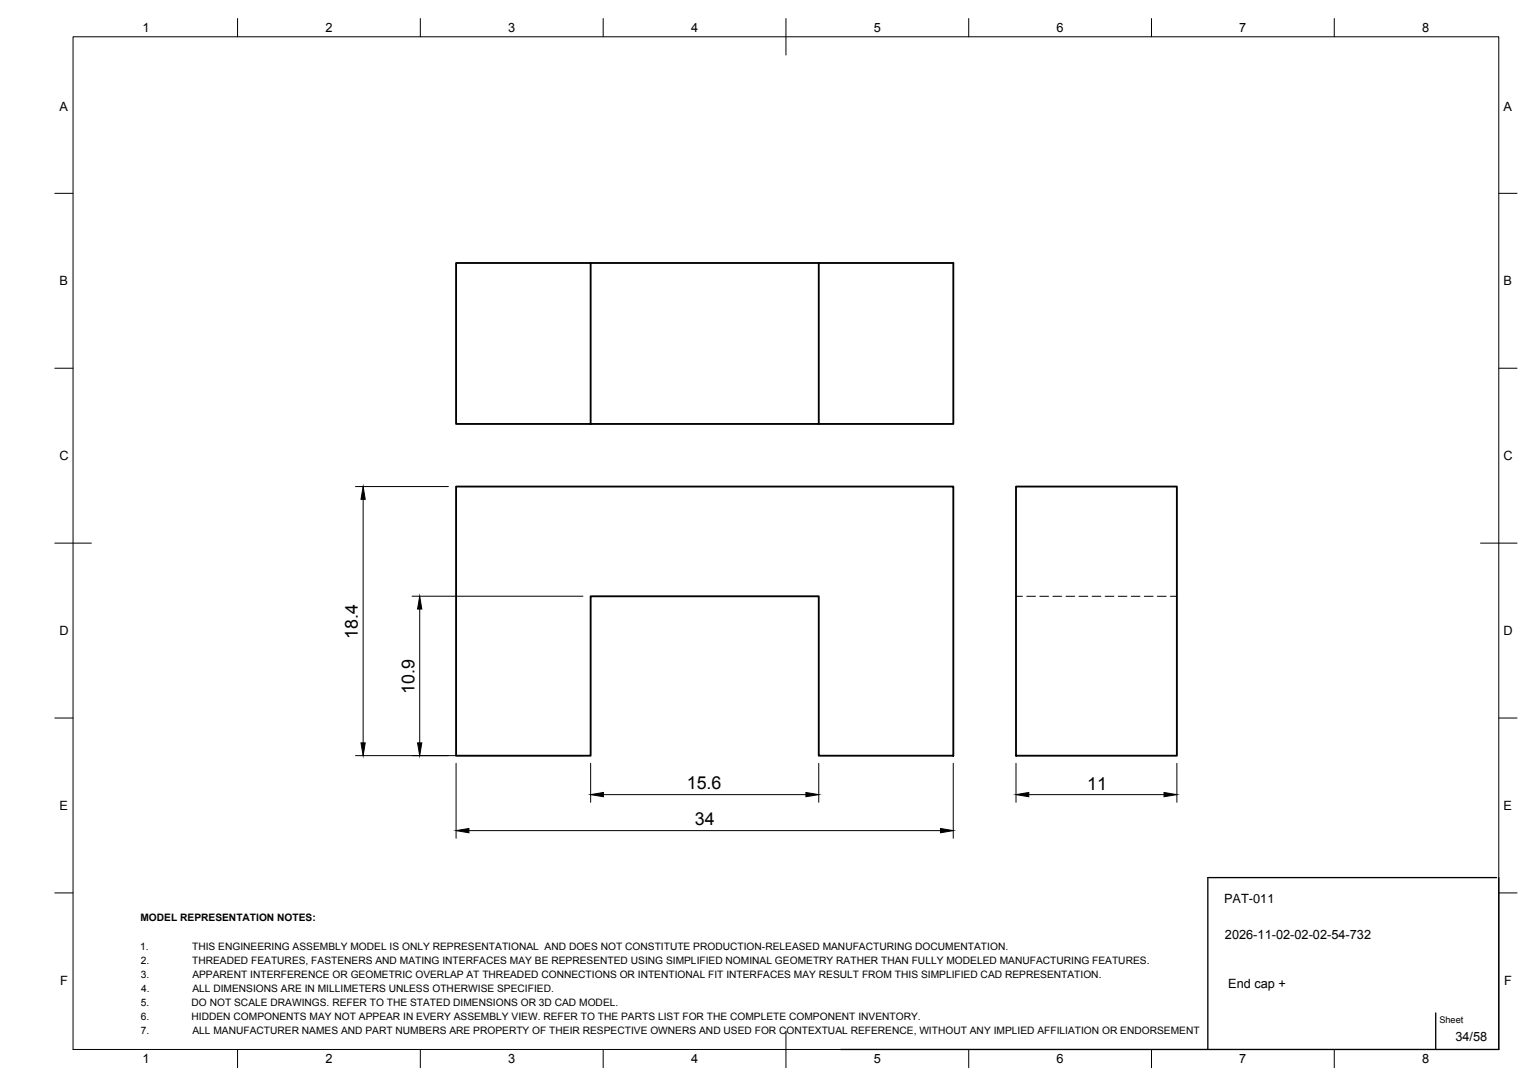
ISO-10303-21;
HEADER;
/* Generated by software containing ST-Developer
 * from STEP Tools, Inc. (www.steptools.com) 
 */

FILE_DESCRIPTION(
/* description */ ('Belt tension measurement rig'),
/* implementation_level */ '2;1');

FILE_NAME(
/* name */ 'End cap +.step',
/* time_stamp */ '2026-10-28T03:24:44-07:00',
/* author */ (''),
/* organization */ (''),
/* preprocessor_version */ 'ST-DEVELOPER v20.2',
/* originating_system */ 'Autodesk Translation Framework v15.17.0.0',
/* authorisation */ '');

FILE_SCHEMA (('AUTOMOTIVE_DESIGN { 1 0 10303 214 3 1 1 }'));
ENDSEC;

DATA;
#10=MECHANICAL_DESIGN_GEOMETRIC_PRESENTATION_REPRESENTATION('',(#728),#23587);
#610=SHAPE_REPRESENTATION_RELATIONSHIP('SRR','None',#23858,#665);
#665=ADVANCED_BREP_SHAPE_REPRESENTATION('',(#798),#23556);
#728=STYLED_ITEM('',(#24204),#798);
#798=MANIFOLD_SOLID_BREP('Body1',#12233);
#1219=PLANE('',#13605);
#1220=PLANE('',#13606);
#1221=PLANE('',#13607);
#1222=PLANE('',#13608);
#1223=PLANE('',#13609);
#1224=PLANE('',#13610);
#1225=PLANE('',#13611);
#1226=PLANE('',#13612);
#1227=PLANE('',#13613);
#1228=PLANE('',#13614);
#1699=FACE_OUTER_BOUND('',#2547,.T.);
#1700=FACE_OUTER_BOUND('',#2548,.T.);
#1701=FACE_OUTER_BOUND('',#2549,.T.);
#1702=FACE_OUTER_BOUND('',#2550,.T.);
#1703=FACE_OUTER_BOUND('',#2551,.T.);
#1704=FACE_OUTER_BOUND('',#2552,.T.);
#1705=FACE_OUTER_BOUND('',#2553,.T.);
#1706=FACE_OUTER_BOUND('',#2554,.T.);
#1707=FACE_OUTER_BOUND('',#2555,.T.);
#1708=FACE_OUTER_BOUND('',#2556,.T.);
#2547=EDGE_LOOP('',(#9506,#9507,#9508,#9509));
#2548=EDGE_LOOP('',(#9510,#9511,#9512,#9513));
#2549=EDGE_LOOP('',(#9514,#9515,#9516,#9517));
#2550=EDGE_LOOP('',(#9518,#9519,#9520,#9521));
#2551=EDGE_LOOP('',(#9522,#9523,#9524,#9525));
#2552=EDGE_LOOP('',(#9526,#9527,#9528,#9529));
#2553=EDGE_LOOP('',(#9530,#9531,#9532,#9533));
#2554=EDGE_LOOP('',(#9534,#9535,#9536,#9537));
#2555=EDGE_LOOP('',(#9538,#9539,#9540,#9541,#9542,#9543,#9544,#9545));
#2556=EDGE_LOOP('',(#9546,#9547,#9548,#9549,#9550,#9551,#9552,#9553));
#3383=LINE('',#20682,#4134);
#3384=LINE('',#20684,#4135);
#3385=LINE('',#20686,#4136);
#3386=LINE('',#20687,#4137);
#3387=LINE('',#20690,#4138);
#3388=LINE('',#20692,#4139);
#3389=LINE('',#20693,#4140);
#3390=LINE('',#20696,#4141);
#3391=LINE('',#20698,#4142);
#3392=LINE('',#20699,#4143);
#3393=LINE('',#20702,#4144);
#3394=LINE('',#20704,#4145);
#3395=LINE('',#20705,#4146);
#3396=LINE('',#20708,#4147);
#3397=LINE('',#20710,#4148);
#3398=LINE('',#20711,#4149);
#3399=LINE('',#20714,#4150);
#3400=LINE('',#20716,#4151);
#3401=LINE('',#20717,#4152);
#3402=LINE('',#20720,#4153);
#3403=LINE('',#20722,#4154);
#3404=LINE('',#20723,#4155);
#3405=LINE('',#20725,#4156);
#3406=LINE('',#20726,#4157);
#4134=VECTOR('',#16392,1.);
#4135=VECTOR('',#16393,1.);
#4136=VECTOR('',#16394,1.);
#4137=VECTOR('',#16395,1.);
#4138=VECTOR('',#16398,1.);
#4139=VECTOR('',#16399,1.);
#4140=VECTOR('',#16400,1.);
#4141=VECTOR('',#16403,1.);
#4142=VECTOR('',#16404,1.);
#4143=VECTOR('',#16405,1.);
#4144=VECTOR('',#16408,1.);
#4145=VECTOR('',#16409,1.);
#4146=VECTOR('',#16410,1.);
#4147=VECTOR('',#16413,1.);
#4148=VECTOR('',#16414,1.);
#4149=VECTOR('',#16415,1.);
#4150=VECTOR('',#16418,1.);
#4151=VECTOR('',#16419,1.);
#4152=VECTOR('',#16420,1.);
#4153=VECTOR('',#16423,1.);
#4154=VECTOR('',#16424,1.);
#4155=VECTOR('',#16425,1.);
#4156=VECTOR('',#16428,1.);
#4157=VECTOR('',#16429,1.);
#5767=VERTEX_POINT('',#20680);
#5768=VERTEX_POINT('',#20681);
#5769=VERTEX_POINT('',#20683);
#5770=VERTEX_POINT('',#20685);
#5771=VERTEX_POINT('',#20689);
#5772=VERTEX_POINT('',#20691);
#5773=VERTEX_POINT('',#20695);
#5774=VERTEX_POINT('',#20697);
#5775=VERTEX_POINT('',#20701);
#5776=VERTEX_POINT('',#20703);
#5777=VERTEX_POINT('',#20707);
#5778=VERTEX_POINT('',#20709);
#5779=VERTEX_POINT('',#20713);
#5780=VERTEX_POINT('',#20715);
#5781=VERTEX_POINT('',#20719);
#5782=VERTEX_POINT('',#20721);
#7112=EDGE_CURVE('',#5767,#5768,#3383,.T.);
#7113=EDGE_CURVE('',#5768,#5769,#3384,.T.);
#7114=EDGE_CURVE('',#5770,#5769,#3385,.T.);
#7115=EDGE_CURVE('',#5767,#5770,#3386,.T.);
#7116=EDGE_CURVE('',#5771,#5767,#3387,.T.);
#7117=EDGE_CURVE('',#5772,#5770,#3388,.T.);
#7118=EDGE_CURVE('',#5771,#5772,#3389,.T.);
#7119=EDGE_CURVE('',#5773,#5771,#3390,.T.);
#7120=EDGE_CURVE('',#5774,#5772,#3391,.T.);
#7121=EDGE_CURVE('',#5773,#5774,#3392,.T.);
#7122=EDGE_CURVE('',#5775,#5773,#3393,.T.);
#7123=EDGE_CURVE('',#5776,#5774,#3394,.T.);
#7124=EDGE_CURVE('',#5775,#5776,#3395,.T.);
#7125=EDGE_CURVE('',#5777,#5775,#3396,.T.);
#7126=EDGE_CURVE('',#5778,#5776,#3397,.T.);
#7127=EDGE_CURVE('',#5777,#5778,#3398,.T.);
#7128=EDGE_CURVE('',#5779,#5777,#3399,.T.);
#7129=EDGE_CURVE('',#5780,#5778,#3400,.T.);
#7130=EDGE_CURVE('',#5779,#5780,#3401,.T.);
#7131=EDGE_CURVE('',#5781,#5779,#3402,.T.);
#7132=EDGE_CURVE('',#5782,#5780,#3403,.T.);
#7133=EDGE_CURVE('',#5781,#5782,#3404,.T.);
#7134=EDGE_CURVE('',#5768,#5781,#3405,.T.);
#7135=EDGE_CURVE('',#5769,#5782,#3406,.T.);
#9506=ORIENTED_EDGE('',*,*,#7112,.T.);
#9507=ORIENTED_EDGE('',*,*,#7113,.T.);
#9508=ORIENTED_EDGE('',*,*,#7114,.F.);
#9509=ORIENTED_EDGE('',*,*,#7115,.F.);
#9510=ORIENTED_EDGE('',*,*,#7116,.T.);
#9511=ORIENTED_EDGE('',*,*,#7115,.T.);
#9512=ORIENTED_EDGE('',*,*,#7117,.F.);
#9513=ORIENTED_EDGE('',*,*,#7118,.F.);
#9514=ORIENTED_EDGE('',*,*,#7119,.T.);
#9515=ORIENTED_EDGE('',*,*,#7118,.T.);
#9516=ORIENTED_EDGE('',*,*,#7120,.F.);
#9517=ORIENTED_EDGE('',*,*,#7121,.F.);
#9518=ORIENTED_EDGE('',*,*,#7122,.T.);
#9519=ORIENTED_EDGE('',*,*,#7121,.T.);
#9520=ORIENTED_EDGE('',*,*,#7123,.F.);
#9521=ORIENTED_EDGE('',*,*,#7124,.F.);
#9522=ORIENTED_EDGE('',*,*,#7125,.T.);
#9523=ORIENTED_EDGE('',*,*,#7124,.T.);
#9524=ORIENTED_EDGE('',*,*,#7126,.F.);
#9525=ORIENTED_EDGE('',*,*,#7127,.F.);
#9526=ORIENTED_EDGE('',*,*,#7128,.T.);
#9527=ORIENTED_EDGE('',*,*,#7127,.T.);
#9528=ORIENTED_EDGE('',*,*,#7129,.F.);
#9529=ORIENTED_EDGE('',*,*,#7130,.F.);
#9530=ORIENTED_EDGE('',*,*,#7131,.T.);
#9531=ORIENTED_EDGE('',*,*,#7130,.T.);
#9532=ORIENTED_EDGE('',*,*,#7132,.F.);
#9533=ORIENTED_EDGE('',*,*,#7133,.F.);
#9534=ORIENTED_EDGE('',*,*,#7134,.T.);
#9535=ORIENTED_EDGE('',*,*,#7133,.T.);
#9536=ORIENTED_EDGE('',*,*,#7135,.F.);
#9537=ORIENTED_EDGE('',*,*,#7113,.F.);
#9538=ORIENTED_EDGE('',*,*,#7135,.T.);
#9539=ORIENTED_EDGE('',*,*,#7132,.T.);
#9540=ORIENTED_EDGE('',*,*,#7129,.T.);
#9541=ORIENTED_EDGE('',*,*,#7126,.T.);
#9542=ORIENTED_EDGE('',*,*,#7123,.T.);
#9543=ORIENTED_EDGE('',*,*,#7120,.T.);
#9544=ORIENTED_EDGE('',*,*,#7117,.T.);
#9545=ORIENTED_EDGE('',*,*,#7114,.T.);
#9546=ORIENTED_EDGE('',*,*,#7134,.F.);
#9547=ORIENTED_EDGE('',*,*,#7112,.F.);
#9548=ORIENTED_EDGE('',*,*,#7116,.F.);
#9549=ORIENTED_EDGE('',*,*,#7119,.F.);
#9550=ORIENTED_EDGE('',*,*,#7122,.F.);
#9551=ORIENTED_EDGE('',*,*,#7125,.F.);
#9552=ORIENTED_EDGE('',*,*,#7128,.F.);
#9553=ORIENTED_EDGE('',*,*,#7131,.F.);
#11840=ADVANCED_FACE('',(#1699),#1219,.T.);
#11841=ADVANCED_FACE('',(#1700),#1220,.T.);
#11842=ADVANCED_FACE('',(#1701),#1221,.T.);
#11843=ADVANCED_FACE('',(#1702),#1222,.T.);
#11844=ADVANCED_FACE('',(#1703),#1223,.T.);
#11845=ADVANCED_FACE('',(#1704),#1224,.T.);
#11846=ADVANCED_FACE('',(#1705),#1225,.T.);
#11847=ADVANCED_FACE('',(#1706),#1226,.T.);
#11848=ADVANCED_FACE('',(#1707),#1227,.T.);
#11849=ADVANCED_FACE('',(#1708),#1228,.F.);
#12233=CLOSED_SHELL('',(#11840,#11841,#11842,#11843,#11844,#11845,#11846,
#11847,#11848,#11849));
#13604=AXIS2_PLACEMENT_3D('',#20678,#16388,#16389);
#13605=AXIS2_PLACEMENT_3D('',#20679,#16390,#16391);
#13606=AXIS2_PLACEMENT_3D('',#20688,#16396,#16397);
#13607=AXIS2_PLACEMENT_3D('',#20694,#16401,#16402);
#13608=AXIS2_PLACEMENT_3D('',#20700,#16406,#16407);
#13609=AXIS2_PLACEMENT_3D('',#20706,#16411,#16412);
#13610=AXIS2_PLACEMENT_3D('',#20712,#16416,#16417);
#13611=AXIS2_PLACEMENT_3D('',#20718,#16421,#16422);
#13612=AXIS2_PLACEMENT_3D('',#20724,#16426,#16427);
#13613=AXIS2_PLACEMENT_3D('',#20727,#16430,#16431);
#13614=AXIS2_PLACEMENT_3D('',#20728,#16432,#16433);
#16388=DIRECTION('axis',(0.,0.,1.));
#16389=DIRECTION('refdir',(1.,0.,0.));
#16390=DIRECTION('center_axis',(0.,0.,1.));
#16391=DIRECTION('ref_axis',(0.,-1.,0.));
#16392=DIRECTION('',(0.,-1.,0.));
#16393=DIRECTION('',(1.,0.,0.));
#16394=DIRECTION('',(0.,-1.,0.));
#16395=DIRECTION('',(1.,0.,0.));
#16396=DIRECTION('center_axis',(0.,1.,0.));
#16397=DIRECTION('ref_axis',(0.,0.,1.));
#16398=DIRECTION('',(0.,0.,1.));
#16399=DIRECTION('',(0.,0.,1.));
#16400=DIRECTION('',(1.,0.,0.));
#16401=DIRECTION('center_axis',(0.,0.,-1.));
#16402=DIRECTION('ref_axis',(0.,1.,0.));
#16403=DIRECTION('',(0.,1.,0.));
#16404=DIRECTION('',(0.,1.,0.));
#16405=DIRECTION('',(1.,0.,0.));
#16406=DIRECTION('center_axis',(0.,-1.,0.));
#16407=DIRECTION('ref_axis',(0.,0.,-1.));
#16408=DIRECTION('',(0.,0.,-1.));
#16409=DIRECTION('',(0.,0.,-1.));
#16410=DIRECTION('',(1.,0.,0.));
#16411=DIRECTION('center_axis',(0.,0.,-1.));
#16412=DIRECTION('ref_axis',(0.,1.,0.));
#16413=DIRECTION('',(0.,1.,0.));
#16414=DIRECTION('',(0.,1.,0.));
#16415=DIRECTION('',(1.,0.,0.));
#16416=DIRECTION('center_axis',(0.,1.,0.));
#16417=DIRECTION('ref_axis',(0.,0.,1.));
#16418=DIRECTION('',(0.,0.,1.));
#16419=DIRECTION('',(0.,0.,1.));
#16420=DIRECTION('',(1.,0.,0.));
#16421=DIRECTION('center_axis',(0.,0.,-1.));
#16422=DIRECTION('ref_axis',(0.,1.,0.));
#16423=DIRECTION('',(0.,1.,0.));
#16424=DIRECTION('',(0.,1.,0.));
#16425=DIRECTION('',(1.,0.,0.));
#16426=DIRECTION('center_axis',(0.,-1.,0.));
#16427=DIRECTION('ref_axis',(0.,0.,-1.));
#16428=DIRECTION('',(0.,0.,-1.));
#16429=DIRECTION('',(0.,0.,-1.));
#16430=DIRECTION('center_axis',(1.,0.,0.));
#16431=DIRECTION('ref_axis',(0.,0.,-1.));
#16432=DIRECTION('center_axis',(1.,0.,0.));
#16433=DIRECTION('ref_axis',(0.,0.,-1.));
#20678=CARTESIAN_POINT('',(0.,0.,0.));
#20679=CARTESIAN_POINT('Origin',(1.97,1.7,2.3));
#20680=CARTESIAN_POINT('',(1.97,1.7,2.3));
#20681=CARTESIAN_POINT('',(1.97,-1.7,2.3));
#20682=CARTESIAN_POINT('',(1.97,1.7,2.3));
#20683=CARTESIAN_POINT('',(3.07,-1.7,2.3));
#20684=CARTESIAN_POINT('',(1.97,-1.7,2.3));
#20685=CARTESIAN_POINT('',(3.07,1.7,2.3));
#20686=CARTESIAN_POINT('',(3.07,1.7,2.3));
#20687=CARTESIAN_POINT('',(1.97,1.7,2.3));
#20688=CARTESIAN_POINT('Origin',(1.97,1.7,0.46));
#20689=CARTESIAN_POINT('',(1.97,1.7,0.46));
#20690=CARTESIAN_POINT('',(1.97,1.7,0.46));
#20691=CARTESIAN_POINT('',(3.07,1.7,0.46));
#20692=CARTESIAN_POINT('',(3.07,1.7,0.46));
#20693=CARTESIAN_POINT('',(1.97,1.7,0.46));
#20694=CARTESIAN_POINT('Origin',(1.97,0.78,0.46));
#20695=CARTESIAN_POINT('',(1.97,0.78,0.46));
#20696=CARTESIAN_POINT('',(1.97,0.78,0.46));
#20697=CARTESIAN_POINT('',(3.07,0.78,0.46));
#20698=CARTESIAN_POINT('',(3.07,0.78,0.46));
#20699=CARTESIAN_POINT('',(1.97,0.78,0.46));
#20700=CARTESIAN_POINT('Origin',(1.97,0.78,1.55));
#20701=CARTESIAN_POINT('',(1.97,0.78,1.55));
#20702=CARTESIAN_POINT('',(1.97,0.78,1.55));
#20703=CARTESIAN_POINT('',(3.07,0.78,1.55));
#20704=CARTESIAN_POINT('',(3.07,0.78,1.55));
#20705=CARTESIAN_POINT('',(1.97,0.78,1.55));
#20706=CARTESIAN_POINT('Origin',(1.97,-0.78,1.55));
#20707=CARTESIAN_POINT('',(1.97,-0.78,1.55));
#20708=CARTESIAN_POINT('',(1.97,-0.78,1.55));
#20709=CARTESIAN_POINT('',(3.07,-0.78,1.55));
#20710=CARTESIAN_POINT('',(3.07,-0.78,1.55));
#20711=CARTESIAN_POINT('',(1.97,-0.78,1.55));
#20712=CARTESIAN_POINT('Origin',(1.97,-0.78,0.46));
#20713=CARTESIAN_POINT('',(1.97,-0.78,0.46));
#20714=CARTESIAN_POINT('',(1.97,-0.78,0.46));
#20715=CARTESIAN_POINT('',(3.07,-0.78,0.46));
#20716=CARTESIAN_POINT('',(3.07,-0.78,0.46));
#20717=CARTESIAN_POINT('',(1.97,-0.78,0.46));
#20718=CARTESIAN_POINT('Origin',(1.97,-1.7,0.46));
#20719=CARTESIAN_POINT('',(1.97,-1.7,0.46));
#20720=CARTESIAN_POINT('',(1.97,-1.7,0.46));
#20721=CARTESIAN_POINT('',(3.07,-1.7,0.46));
#20722=CARTESIAN_POINT('',(3.07,-1.7,0.46));
#20723=CARTESIAN_POINT('',(1.97,-1.7,0.46));
#20724=CARTESIAN_POINT('Origin',(1.97,-1.7,2.3));
#20725=CARTESIAN_POINT('',(1.97,-1.7,2.3));
#20726=CARTESIAN_POINT('',(3.07,-1.7,2.3));
#20727=CARTESIAN_POINT('Origin',(3.07,0.,1.38));
#20728=CARTESIAN_POINT('Origin',(1.97,0.,1.38));
#23491=UNCERTAINTY_MEASURE_WITH_UNIT(LENGTH_MEASURE(0.001),#23588,
'DISTANCE_ACCURACY_VALUE',
'Maximum model space distance between geometric entities at asserted c
onnectivities');
#23522=UNCERTAINTY_MEASURE_WITH_UNIT(LENGTH_MEASURE(0.001),#23588,
'DISTANCE_ACCURACY_VALUE',
'Maximum model space distance between geometric entities at asserted c
onnectivities');
#23556=(
GEOMETRIC_REPRESENTATION_CONTEXT(3)
GLOBAL_UNCERTAINTY_ASSIGNED_CONTEXT((#23491))
GLOBAL_UNIT_ASSIGNED_CONTEXT((#23588,#23590,#23591))
REPRESENTATION_CONTEXT('','3D')
);
#23587=(
GEOMETRIC_REPRESENTATION_CONTEXT(3)
GLOBAL_UNCERTAINTY_ASSIGNED_CONTEXT((#23522))
GLOBAL_UNIT_ASSIGNED_CONTEXT((#23588,#23590,#23591))
REPRESENTATION_CONTEXT('','3D')
);
#23588=(
LENGTH_UNIT()
NAMED_UNIT(*)
SI_UNIT(.CENTI.,.METRE.)
);
#23590=(
NAMED_UNIT(*)
PLANE_ANGLE_UNIT()
SI_UNIT($,.RADIAN.)
);
#23591=(
NAMED_UNIT(*)
SI_UNIT($,.STERADIAN.)
SOLID_ANGLE_UNIT()
);
#23625=SHAPE_DEFINITION_REPRESENTATION(#23694,#23858);
#23694=PRODUCT_DEFINITION_SHAPE('',$,#23923);
#23858=SHAPE_REPRESENTATION('',(#13604),#23556);
#23889=PRODUCT_DEFINITION_CONTEXT('part definition',#24083,'design');
#23923=PRODUCT_DEFINITION('End cap +','End cap +',#23987,#23889);
#23987=PRODUCT_DEFINITION_FORMATION('',$,#24118);
#24083=APPLICATION_CONTEXT(
'Core Data for Automotive Mechanical Design Process');
#24084=PRODUCT_CONTEXT('part definition',#24083,'mechanical');
#24118=PRODUCT('End cap +','End cap +','End cap +',(#24084));
#24198=COLOUR_RGB('Sky Blue',0.24,0.69,0.87);
#24199=FILL_AREA_STYLE_COLOUR('',#24198);
#24200=FILL_AREA_STYLE('',(#24199));
#24201=SURFACE_STYLE_FILL_AREA(#24200);
#24202=SURFACE_SIDE_STYLE('',(#24201));
#24203=SURFACE_STYLE_USAGE(.BOTH.,#24202);
#24204=PRESENTATION_STYLE_ASSIGNMENT((#24203));
ENDSEC;
END-ISO-10303-21;
